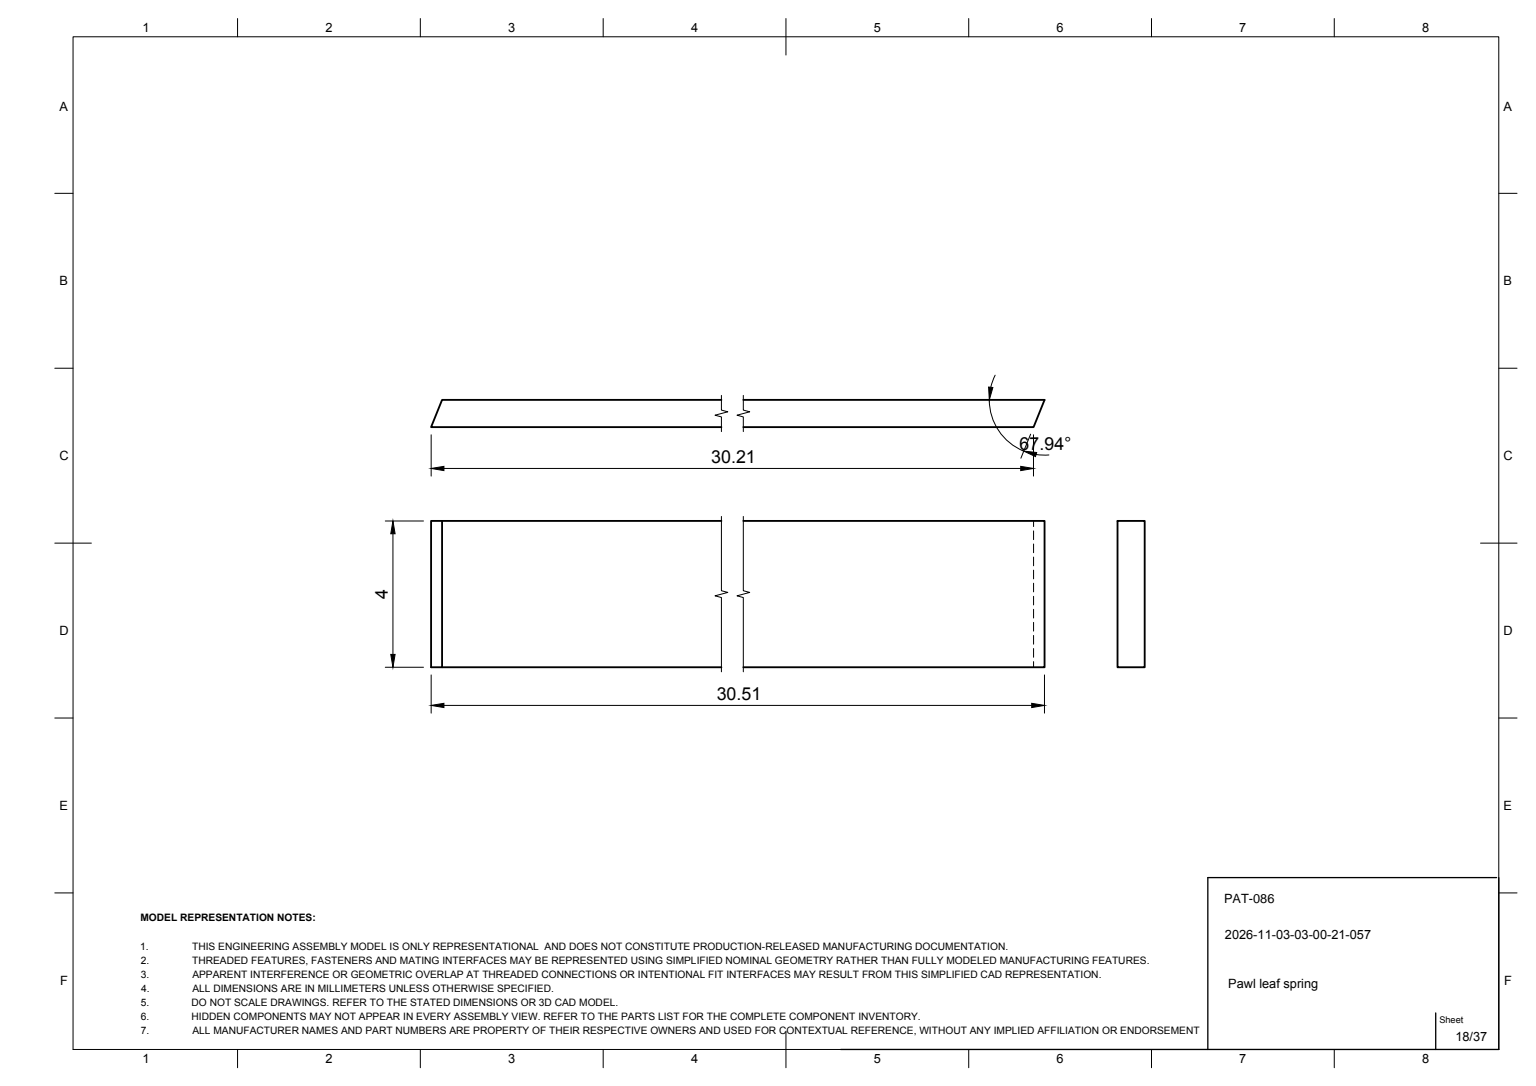
ISO-10303-21;
HEADER;
/* Generated by software containing ST-Developer
 * from STEP Tools, Inc. (www.steptools.com) 
 */

FILE_DESCRIPTION(
/* description */ ('Ratchet and pawl hand winch drum'),
/* implementation_level */ '2;1');

FILE_NAME(
/* name */ 'Pawl leaf spring.step',
/* time_stamp */ '2026-10-27T12:42:58-07:00',
/* author */ (''),
/* organization */ (''),
/* preprocessor_version */ 'ST-DEVELOPER v20.2',
/* originating_system */ 'Autodesk Translation Framework v15.17.0.0',
/* authorisation */ '');

FILE_SCHEMA (('AUTOMOTIVE_DESIGN { 1 0 10303 214 3 1 1 }'));
ENDSEC;

DATA;
#10=MECHANICAL_DESIGN_GEOMETRIC_PRESENTATION_REPRESENTATION('',(#402),#11801);
#334=SHAPE_REPRESENTATION_RELATIONSHIP('SRR','None',#11960,#368);
#368=ADVANCED_BREP_SHAPE_REPRESENTATION('',(#437),#11777);
#402=STYLED_ITEM('',(#12213),#437);
#437=MANIFOLD_SOLID_BREP('Body1',#6279);
#666=PLANE('',#6904);
#667=PLANE('',#6905);
#668=PLANE('',#6906);
#669=PLANE('',#6907);
#670=PLANE('',#6908);
#671=PLANE('',#6909);
#953=FACE_OUTER_BOUND('',#1382,.T.);
#954=FACE_OUTER_BOUND('',#1383,.T.);
#955=FACE_OUTER_BOUND('',#1384,.T.);
#956=FACE_OUTER_BOUND('',#1385,.T.);
#957=FACE_OUTER_BOUND('',#1386,.T.);
#958=FACE_OUTER_BOUND('',#1387,.T.);
#1382=EDGE_LOOP('',(#4703,#4704,#4705,#4706));
#1383=EDGE_LOOP('',(#4707,#4708,#4709,#4710));
#1384=EDGE_LOOP('',(#4711,#4712,#4713,#4714));
#1385=EDGE_LOOP('',(#4715,#4716,#4717,#4718));
#1386=EDGE_LOOP('',(#4719,#4720,#4721,#4722));
#1387=EDGE_LOOP('',(#4723,#4724,#4725,#4726));
#1829=LINE('',#9739,#2340);
#1830=LINE('',#9741,#2341);
#1831=LINE('',#9743,#2342);
#1832=LINE('',#9744,#2343);
#1833=LINE('',#9747,#2344);
#1834=LINE('',#9749,#2345);
#1835=LINE('',#9750,#2346);
#1836=LINE('',#9753,#2347);
#1837=LINE('',#9755,#2348);
#1838=LINE('',#9756,#2349);
#1839=LINE('',#9758,#2350);
#1840=LINE('',#9759,#2351);
#2340=VECTOR('',#7942,1.);
#2341=VECTOR('',#7943,1.);
#2342=VECTOR('',#7944,1.);
#2343=VECTOR('',#7945,1.);
#2344=VECTOR('',#7948,1.);
#2345=VECTOR('',#7949,1.);
#2346=VECTOR('',#7950,1.);
#2347=VECTOR('',#7953,1.);
#2348=VECTOR('',#7954,1.);
#2349=VECTOR('',#7955,1.);
#2350=VECTOR('',#7958,1.);
#2351=VECTOR('',#7959,1.);
#3094=VERTEX_POINT('',#9737);
#3095=VERTEX_POINT('',#9738);
#3096=VERTEX_POINT('',#9740);
#3097=VERTEX_POINT('',#9742);
#3098=VERTEX_POINT('',#9746);
#3099=VERTEX_POINT('',#9748);
#3100=VERTEX_POINT('',#9752);
#3101=VERTEX_POINT('',#9754);
#3695=EDGE_CURVE('',#3094,#3095,#1829,.T.);
#3696=EDGE_CURVE('',#3094,#3096,#1830,.T.);
#3697=EDGE_CURVE('',#3097,#3096,#1831,.T.);
#3698=EDGE_CURVE('',#3095,#3097,#1832,.T.);
#3699=EDGE_CURVE('',#3095,#3098,#1833,.T.);
#3700=EDGE_CURVE('',#3099,#3097,#1834,.T.);
#3701=EDGE_CURVE('',#3098,#3099,#1835,.T.);
#3702=EDGE_CURVE('',#3098,#3100,#1836,.T.);
#3703=EDGE_CURVE('',#3101,#3099,#1837,.T.);
#3704=EDGE_CURVE('',#3100,#3101,#1838,.T.);
#3705=EDGE_CURVE('',#3100,#3094,#1839,.T.);
#3706=EDGE_CURVE('',#3096,#3101,#1840,.T.);
#4703=ORIENTED_EDGE('',*,*,#3695,.F.);
#4704=ORIENTED_EDGE('',*,*,#3696,.T.);
#4705=ORIENTED_EDGE('',*,*,#3697,.F.);
#4706=ORIENTED_EDGE('',*,*,#3698,.F.);
#4707=ORIENTED_EDGE('',*,*,#3699,.F.);
#4708=ORIENTED_EDGE('',*,*,#3698,.T.);
#4709=ORIENTED_EDGE('',*,*,#3700,.F.);
#4710=ORIENTED_EDGE('',*,*,#3701,.F.);
#4711=ORIENTED_EDGE('',*,*,#3702,.F.);
#4712=ORIENTED_EDGE('',*,*,#3701,.T.);
#4713=ORIENTED_EDGE('',*,*,#3703,.F.);
#4714=ORIENTED_EDGE('',*,*,#3704,.F.);
#4715=ORIENTED_EDGE('',*,*,#3705,.F.);
#4716=ORIENTED_EDGE('',*,*,#3704,.T.);
#4717=ORIENTED_EDGE('',*,*,#3706,.F.);
#4718=ORIENTED_EDGE('',*,*,#3696,.F.);
#4719=ORIENTED_EDGE('',*,*,#3706,.T.);
#4720=ORIENTED_EDGE('',*,*,#3703,.T.);
#4721=ORIENTED_EDGE('',*,*,#3700,.T.);
#4722=ORIENTED_EDGE('',*,*,#3697,.T.);
#4723=ORIENTED_EDGE('',*,*,#3705,.T.);
#4724=ORIENTED_EDGE('',*,*,#3695,.T.);
#4725=ORIENTED_EDGE('',*,*,#3699,.T.);
#4726=ORIENTED_EDGE('',*,*,#3702,.T.);
#6023=ADVANCED_FACE('',(#953),#666,.T.);
#6024=ADVANCED_FACE('',(#954),#667,.T.);
#6025=ADVANCED_FACE('',(#955),#668,.T.);
#6026=ADVANCED_FACE('',(#956),#669,.T.);
#6027=ADVANCED_FACE('',(#957),#670,.T.);
#6028=ADVANCED_FACE('',(#958),#671,.F.);
#6279=CLOSED_SHELL('',(#6023,#6024,#6025,#6026,#6027,#6028));
#6903=AXIS2_PLACEMENT_3D('',#9735,#7938,#7939);
#6904=AXIS2_PLACEMENT_3D('',#9736,#7940,#7941);
#6905=AXIS2_PLACEMENT_3D('',#9745,#7946,#7947);
#6906=AXIS2_PLACEMENT_3D('',#9751,#7951,#7952);
#6907=AXIS2_PLACEMENT_3D('',#9757,#7956,#7957);
#6908=AXIS2_PLACEMENT_3D('',#9760,#7960,#7961);
#6909=AXIS2_PLACEMENT_3D('',#9761,#7962,#7963);
#7938=DIRECTION('axis',(0.,0.,1.));
#7939=DIRECTION('refdir',(1.,0.,0.));
#7940=DIRECTION('center_axis',(-0.926809259863616,0.,-0.37553241648499));
#7941=DIRECTION('ref_axis',(-0.37553241648499,0.,0.926809259863616));
#7942=DIRECTION('',(0.37553241648499,0.,-0.926809259863616));
#7943=DIRECTION('',(0.,1.,0.));
#7944=DIRECTION('',(-0.37553241648499,0.,0.926809259863616));
#7945=DIRECTION('',(0.,1.,0.));
#7946=DIRECTION('center_axis',(0.,0.,-1.));
#7947=DIRECTION('ref_axis',(-1.,0.,0.));
#7948=DIRECTION('',(1.,0.,0.));
#7949=DIRECTION('',(-1.,0.,0.));
#7950=DIRECTION('',(0.,1.,0.));
#7951=DIRECTION('center_axis',(0.926809259863616,0.,0.37553241648499));
#7952=DIRECTION('ref_axis',(0.37553241648499,0.,-0.926809259863616));
#7953=DIRECTION('',(-0.37553241648499,0.,0.926809259863616));
#7954=DIRECTION('',(0.37553241648499,0.,-0.926809259863616));
#7955=DIRECTION('',(0.,1.,0.));
#7956=DIRECTION('center_axis',(0.,0.,1.));
#7957=DIRECTION('ref_axis',(1.,0.,0.));
#7958=DIRECTION('',(-1.,0.,0.));
#7959=DIRECTION('',(1.,0.,0.));
#7960=DIRECTION('center_axis',(0.,1.,0.));
#7961=DIRECTION('ref_axis',(0.,0.,1.));
#7962=DIRECTION('center_axis',(0.,1.,0.));
#7963=DIRECTION('ref_axis',(1.,0.,0.));
#9735=CARTESIAN_POINT('',(0.,0.,0.));
#9736=CARTESIAN_POINT('Origin',(7.9,-3.4,6.5));
#9737=CARTESIAN_POINT('',(6.76547231270358,-3.4,9.3));
#9738=CARTESIAN_POINT('',(7.9,-3.4,6.5));
#9739=CARTESIAN_POINT('',(6.76547231270358,-3.4,9.3));
#9740=CARTESIAN_POINT('',(6.76547231270358,-3.,9.3));
#9741=CARTESIAN_POINT('',(6.76547231270358,-3.4,9.3));
#9742=CARTESIAN_POINT('',(7.9,-3.,6.5));
#9743=CARTESIAN_POINT('',(6.76547231270358,-3.,9.3));
#9744=CARTESIAN_POINT('',(7.9,-3.4,6.5));
#9745=CARTESIAN_POINT('Origin',(7.98,-3.4,6.5));
#9746=CARTESIAN_POINT('',(7.98,-3.4,6.5));
#9747=CARTESIAN_POINT('',(7.9,-3.4,6.5));
#9748=CARTESIAN_POINT('',(7.98,-3.,6.5));
#9749=CARTESIAN_POINT('',(7.9,-3.,6.5));
#9750=CARTESIAN_POINT('',(7.98,-3.4,6.5));
#9751=CARTESIAN_POINT('Origin',(6.84547231270358,-3.4,9.3));
#9752=CARTESIAN_POINT('',(6.84547231270358,-3.4,9.3));
#9753=CARTESIAN_POINT('',(7.98,-3.4,6.5));
#9754=CARTESIAN_POINT('',(6.84547231270358,-3.,9.3));
#9755=CARTESIAN_POINT('',(7.98,-3.,6.5));
#9756=CARTESIAN_POINT('',(6.84547231270358,-3.4,9.3));
#9757=CARTESIAN_POINT('Origin',(6.76547231270358,-3.4,9.3));
#9758=CARTESIAN_POINT('',(6.84547231270358,-3.4,9.3));
#9759=CARTESIAN_POINT('',(6.84547231270358,-3.,9.3));
#9760=CARTESIAN_POINT('Origin',(7.37273615635179,-3.,7.9));
#9761=CARTESIAN_POINT('Origin',(7.37273615635179,-3.4,7.9));
#11737=UNCERTAINTY_MEASURE_WITH_UNIT(LENGTH_MEASURE(0.001),#11802,
'DISTANCE_ACCURACY_VALUE',
'Maximum model space distance between geometric entities at asserted c
onnectivities');
#11761=UNCERTAINTY_MEASURE_WITH_UNIT(LENGTH_MEASURE(0.001),#11802,
'DISTANCE_ACCURACY_VALUE',
'Maximum model space distance between geometric entities at asserted c
onnectivities');
#11777=(
GEOMETRIC_REPRESENTATION_CONTEXT(3)
GLOBAL_UNCERTAINTY_ASSIGNED_CONTEXT((#11737))
GLOBAL_UNIT_ASSIGNED_CONTEXT((#11802,#11804,#11805))
REPRESENTATION_CONTEXT('','3D')
);
#11801=(
GEOMETRIC_REPRESENTATION_CONTEXT(3)
GLOBAL_UNCERTAINTY_ASSIGNED_CONTEXT((#11761))
GLOBAL_UNIT_ASSIGNED_CONTEXT((#11802,#11804,#11805))
REPRESENTATION_CONTEXT('','3D')
);
#11802=(
LENGTH_UNIT()
NAMED_UNIT(*)
SI_UNIT(.CENTI.,.METRE.)
);
#11804=(
NAMED_UNIT(*)
PLANE_ANGLE_UNIT()
SI_UNIT($,.RADIAN.)
);
#11805=(
NAMED_UNIT(*)
SI_UNIT($,.STERADIAN.)
SOLID_ANGLE_UNIT()
);
#11821=SHAPE_DEFINITION_REPRESENTATION(#11860,#11960);
#11860=PRODUCT_DEFINITION_SHAPE('',$,#12000);
#11960=SHAPE_REPRESENTATION('',(#6903),#11777);
#11984=PRODUCT_DEFINITION_CONTEXT('part definition',#12103,'design');
#12000=PRODUCT_DEFINITION('Pawl leaf spring','Pawl leaf spring',#12039,
#11984);
#12039=PRODUCT_DEFINITION_FORMATION('',$,#12120);
#12103=APPLICATION_CONTEXT(
'Core Data for Automotive Mechanical Design Process');
#12104=PRODUCT_CONTEXT('part definition',#12103,'mechanical');
#12120=PRODUCT('Pawl leaf spring','Pawl leaf spring','Pawl leaf spring',
(#12104));
#12207=COLOUR_RGB('Grey',0.48,0.52,0.57);
#12208=FILL_AREA_STYLE_COLOUR('',#12207);
#12209=FILL_AREA_STYLE('',(#12208));
#12210=SURFACE_STYLE_FILL_AREA(#12209);
#12211=SURFACE_SIDE_STYLE('',(#12210));
#12212=SURFACE_STYLE_USAGE(.BOTH.,#12211);
#12213=PRESENTATION_STYLE_ASSIGNMENT((#12212));
ENDSEC;
END-ISO-10303-21;
